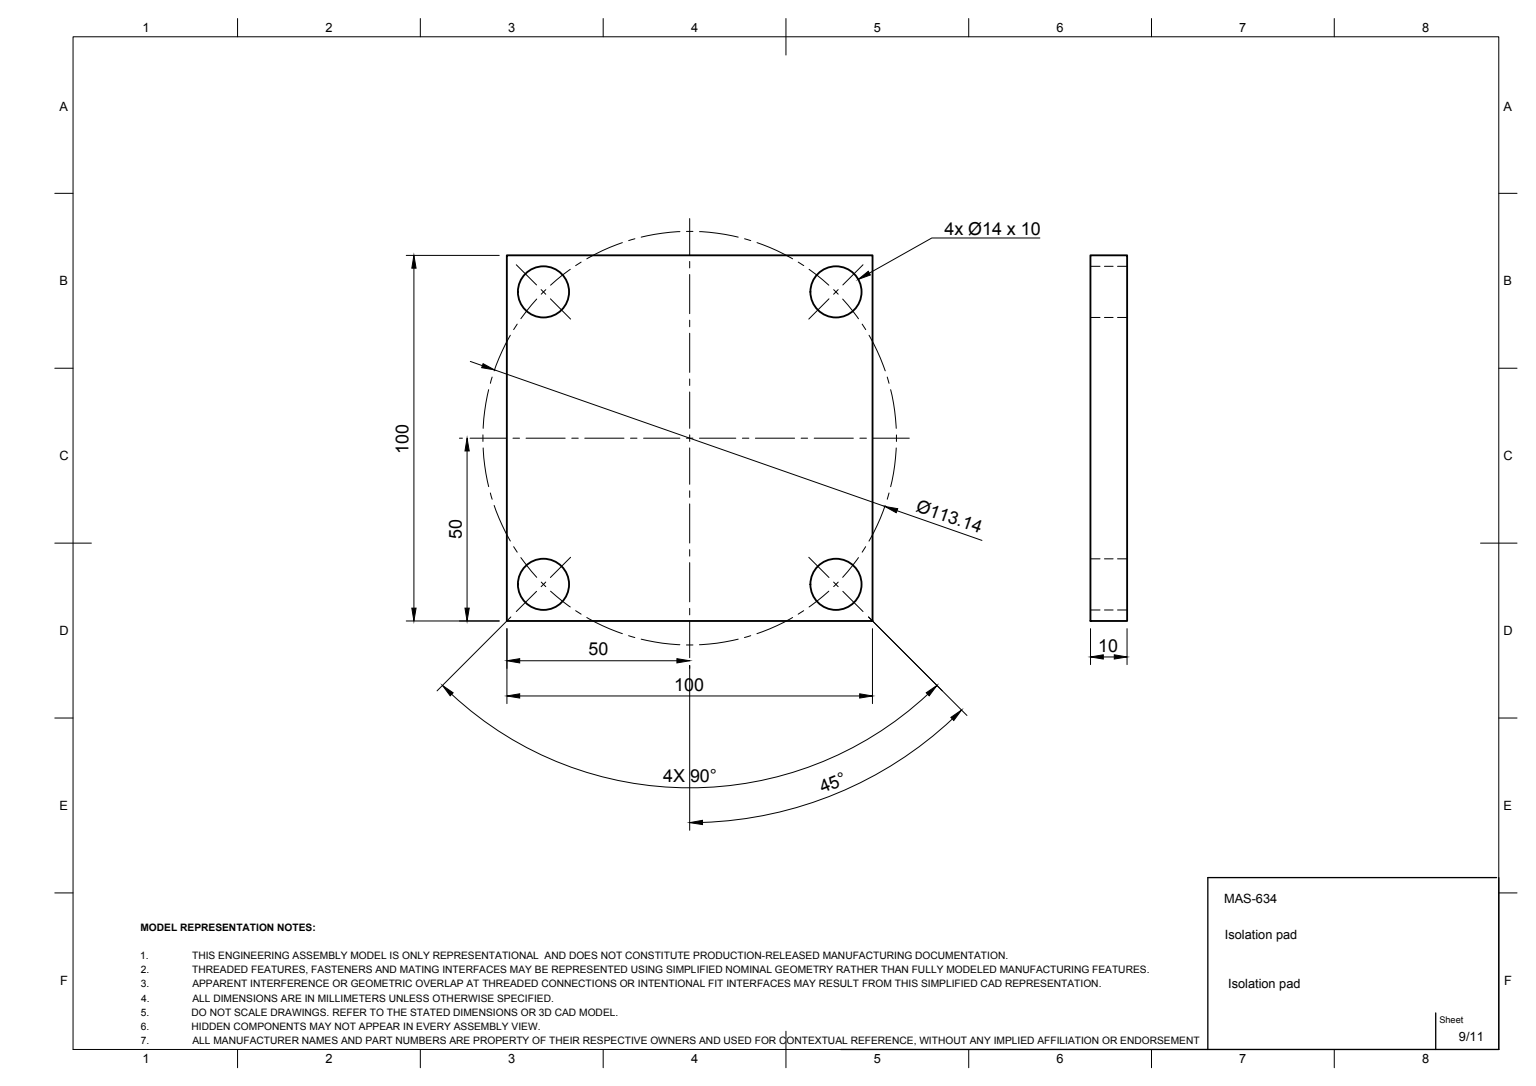
ISO-10303-21;
HEADER;
/* Generated by software containing ST-Developer
 * from STEP Tools, Inc. (www.steptools.com) 
 */

FILE_DESCRIPTION(
/* description */ ('Independent AHU equipment rack. Nominal800x600 frame on1000long40squa
re aluminum posts; two removable notched shelves; welded perimeter/cro
ss rails and rear gussets; two mounting channels; four isolation pads 
and anchor-ready feet. Imported native extrusion library retained and 
cut-length parameters customized per family. Shelf hardware uses model
ed M6 rivet nuts and screws. Weld design, floor anchors and load ratin
g require engineering selection.'),
/* implementation_level */ '2;1');

FILE_NAME(
/* name */ 'Isolation pad.step',
/* time_stamp */ '2026-11-07T19:04:45-08:00',
/* author */ (''),
/* organization */ (''),
/* preprocessor_version */ 'ST-DEVELOPER v20.2',
/* originating_system */ 'Autodesk Translation Framework v15.17.0.0',
/* authorisation */ '');

FILE_SCHEMA (('AUTOMOTIVE_DESIGN { 1 0 10303 214 3 1 1 }'));
ENDSEC;

DATA;
#10=MECHANICAL_DESIGN_GEOMETRIC_PRESENTATION_REPRESENTATION('',(#341),#9777);
#319=SHAPE_REPRESENTATION_RELATIONSHIP('SRR','None',#9863,#330);
#330=ADVANCED_BREP_SHAPE_REPRESENTATION('',(#352),#9772);
#341=STYLED_ITEM('',(#9926),#352);
#352=MANIFOLD_SOLID_BREP('Body1',#3846);
#395=FACE_BOUND('',#855,.T.);
#396=FACE_BOUND('',#856,.T.);
#397=FACE_BOUND('',#857,.T.);
#398=FACE_BOUND('',#858,.T.);
#399=FACE_BOUND('',#860,.T.);
#400=FACE_BOUND('',#861,.T.);
#401=FACE_BOUND('',#862,.T.);
#402=FACE_BOUND('',#863,.T.);
#470=PLANE('',#4197);
#471=PLANE('',#4198);
#472=PLANE('',#4199);
#473=PLANE('',#4200);
#474=PLANE('',#4201);
#475=PLANE('',#4202);
#610=FACE_OUTER_BOUND('',#846,.T.);
#611=FACE_OUTER_BOUND('',#847,.T.);
#612=FACE_OUTER_BOUND('',#848,.T.);
#613=FACE_OUTER_BOUND('',#849,.T.);
#614=FACE_OUTER_BOUND('',#850,.T.);
#615=FACE_OUTER_BOUND('',#851,.T.);
#616=FACE_OUTER_BOUND('',#852,.T.);
#617=FACE_OUTER_BOUND('',#853,.T.);
#618=FACE_OUTER_BOUND('',#854,.T.);
#619=FACE_OUTER_BOUND('',#859,.T.);
#846=EDGE_LOOP('',(#3091,#3092,#3093,#3094));
#847=EDGE_LOOP('',(#3095,#3096,#3097,#3098));
#848=EDGE_LOOP('',(#3099,#3100,#3101,#3102));
#849=EDGE_LOOP('',(#3103,#3104,#3105,#3106));
#850=EDGE_LOOP('',(#3107,#3108,#3109,#3110));
#851=EDGE_LOOP('',(#3111,#3112,#3113,#3114));
#852=EDGE_LOOP('',(#3115,#3116,#3117,#3118));
#853=EDGE_LOOP('',(#3119,#3120,#3121,#3122));
#854=EDGE_LOOP('',(#3123,#3124,#3125,#3126));
#855=EDGE_LOOP('',(#3127));
#856=EDGE_LOOP('',(#3128));
#857=EDGE_LOOP('',(#3129));
#858=EDGE_LOOP('',(#3130));
#859=EDGE_LOOP('',(#3131,#3132,#3133,#3134));
#860=EDGE_LOOP('',(#3135));
#861=EDGE_LOOP('',(#3136));
#862=EDGE_LOOP('',(#3137));
#863=EDGE_LOOP('',(#3138));
#1143=LINE('',#6003,#1436);
#1144=LINE('',#6009,#1437);
#1145=LINE('',#6015,#1438);
#1146=LINE('',#6021,#1439);
#1147=LINE('',#6026,#1440);
#1148=LINE('',#6028,#1441);
#1149=LINE('',#6030,#1442);
#1150=LINE('',#6031,#1443);
#1151=LINE('',#6034,#1444);
#1152=LINE('',#6036,#1445);
#1153=LINE('',#6037,#1446);
#1154=LINE('',#6040,#1447);
#1155=LINE('',#6042,#1448);
#1156=LINE('',#6043,#1449);
#1157=LINE('',#6045,#1450);
#1158=LINE('',#6046,#1451);
#1436=VECTOR('',#4972,7.);
#1437=VECTOR('',#4979,7.);
#1438=VECTOR('',#4986,7.);
#1439=VECTOR('',#4993,7.);
#1440=VECTOR('',#4998,10.);
#1441=VECTOR('',#4999,10.);
#1442=VECTOR('',#5000,10.);
#1443=VECTOR('',#5001,10.);
#1444=VECTOR('',#5004,10.);
#1445=VECTOR('',#5005,10.);
#1446=VECTOR('',#5006,10.);
#1447=VECTOR('',#5009,10.);
#1448=VECTOR('',#5010,10.);
#1449=VECTOR('',#5011,10.);
#1450=VECTOR('',#5014,10.);
#1451=VECTOR('',#5015,10.);
#1633=CIRCLE('',#4186,7.);
#1634=CIRCLE('',#4187,7.);
#1635=CIRCLE('',#4189,7.);
#1636=CIRCLE('',#4190,7.);
#1637=CIRCLE('',#4192,7.);
#1638=CIRCLE('',#4193,7.);
#1639=CIRCLE('',#4195,7.);
#1640=CIRCLE('',#4196,7.);
#1852=VERTEX_POINT('',#6000);
#1853=VERTEX_POINT('',#6002);
#1854=VERTEX_POINT('',#6006);
#1855=VERTEX_POINT('',#6008);
#1856=VERTEX_POINT('',#6012);
#1857=VERTEX_POINT('',#6014);
#1858=VERTEX_POINT('',#6018);
#1859=VERTEX_POINT('',#6020);
#1860=VERTEX_POINT('',#6024);
#1861=VERTEX_POINT('',#6025);
#1862=VERTEX_POINT('',#6027);
#1863=VERTEX_POINT('',#6029);
#1864=VERTEX_POINT('',#6033);
#1865=VERTEX_POINT('',#6035);
#1866=VERTEX_POINT('',#6039);
#1867=VERTEX_POINT('',#6041);
#2290=EDGE_CURVE('',#1852,#1852,#1633,.T.);
#2291=EDGE_CURVE('',#1852,#1853,#1143,.T.);
#2292=EDGE_CURVE('',#1853,#1853,#1634,.T.);
#2293=EDGE_CURVE('',#1854,#1854,#1635,.T.);
#2294=EDGE_CURVE('',#1854,#1855,#1144,.T.);
#2295=EDGE_CURVE('',#1855,#1855,#1636,.T.);
#2296=EDGE_CURVE('',#1856,#1856,#1637,.T.);
#2297=EDGE_CURVE('',#1856,#1857,#1145,.T.);
#2298=EDGE_CURVE('',#1857,#1857,#1638,.T.);
#2299=EDGE_CURVE('',#1858,#1858,#1639,.T.);
#2300=EDGE_CURVE('',#1858,#1859,#1146,.T.);
#2301=EDGE_CURVE('',#1859,#1859,#1640,.T.);
#2302=EDGE_CURVE('',#1860,#1861,#1147,.T.);
#2303=EDGE_CURVE('',#1861,#1862,#1148,.T.);
#2304=EDGE_CURVE('',#1863,#1862,#1149,.T.);
#2305=EDGE_CURVE('',#1860,#1863,#1150,.T.);
#2306=EDGE_CURVE('',#1864,#1860,#1151,.T.);
#2307=EDGE_CURVE('',#1865,#1863,#1152,.T.);
#2308=EDGE_CURVE('',#1864,#1865,#1153,.T.);
#2309=EDGE_CURVE('',#1866,#1864,#1154,.T.);
#2310=EDGE_CURVE('',#1867,#1865,#1155,.T.);
#2311=EDGE_CURVE('',#1866,#1867,#1156,.T.);
#2312=EDGE_CURVE('',#1861,#1866,#1157,.T.);
#2313=EDGE_CURVE('',#1862,#1867,#1158,.T.);
#3091=ORIENTED_EDGE('',*,*,#2290,.F.);
#3092=ORIENTED_EDGE('',*,*,#2291,.T.);
#3093=ORIENTED_EDGE('',*,*,#2292,.F.);
#3094=ORIENTED_EDGE('',*,*,#2291,.F.);
#3095=ORIENTED_EDGE('',*,*,#2293,.F.);
#3096=ORIENTED_EDGE('',*,*,#2294,.T.);
#3097=ORIENTED_EDGE('',*,*,#2295,.F.);
#3098=ORIENTED_EDGE('',*,*,#2294,.F.);
#3099=ORIENTED_EDGE('',*,*,#2296,.F.);
#3100=ORIENTED_EDGE('',*,*,#2297,.T.);
#3101=ORIENTED_EDGE('',*,*,#2298,.F.);
#3102=ORIENTED_EDGE('',*,*,#2297,.F.);
#3103=ORIENTED_EDGE('',*,*,#2299,.F.);
#3104=ORIENTED_EDGE('',*,*,#2300,.T.);
#3105=ORIENTED_EDGE('',*,*,#2301,.F.);
#3106=ORIENTED_EDGE('',*,*,#2300,.F.);
#3107=ORIENTED_EDGE('',*,*,#2302,.T.);
#3108=ORIENTED_EDGE('',*,*,#2303,.T.);
#3109=ORIENTED_EDGE('',*,*,#2304,.F.);
#3110=ORIENTED_EDGE('',*,*,#2305,.F.);
#3111=ORIENTED_EDGE('',*,*,#2306,.T.);
#3112=ORIENTED_EDGE('',*,*,#2305,.T.);
#3113=ORIENTED_EDGE('',*,*,#2307,.F.);
#3114=ORIENTED_EDGE('',*,*,#2308,.F.);
#3115=ORIENTED_EDGE('',*,*,#2309,.T.);
#3116=ORIENTED_EDGE('',*,*,#2308,.T.);
#3117=ORIENTED_EDGE('',*,*,#2310,.F.);
#3118=ORIENTED_EDGE('',*,*,#2311,.F.);
#3119=ORIENTED_EDGE('',*,*,#2312,.T.);
#3120=ORIENTED_EDGE('',*,*,#2311,.T.);
#3121=ORIENTED_EDGE('',*,*,#2313,.F.);
#3122=ORIENTED_EDGE('',*,*,#2303,.F.);
#3123=ORIENTED_EDGE('',*,*,#2313,.T.);
#3124=ORIENTED_EDGE('',*,*,#2310,.T.);
#3125=ORIENTED_EDGE('',*,*,#2307,.T.);
#3126=ORIENTED_EDGE('',*,*,#2304,.T.);
#3127=ORIENTED_EDGE('',*,*,#2290,.T.);
#3128=ORIENTED_EDGE('',*,*,#2293,.T.);
#3129=ORIENTED_EDGE('',*,*,#2296,.T.);
#3130=ORIENTED_EDGE('',*,*,#2299,.T.);
#3131=ORIENTED_EDGE('',*,*,#2312,.F.);
#3132=ORIENTED_EDGE('',*,*,#2302,.F.);
#3133=ORIENTED_EDGE('',*,*,#2306,.F.);
#3134=ORIENTED_EDGE('',*,*,#2309,.F.);
#3135=ORIENTED_EDGE('',*,*,#2292,.T.);
#3136=ORIENTED_EDGE('',*,*,#2295,.T.);
#3137=ORIENTED_EDGE('',*,*,#2298,.T.);
#3138=ORIENTED_EDGE('',*,*,#2301,.T.);
#3589=CYLINDRICAL_SURFACE('',#4185,7.);
#3590=CYLINDRICAL_SURFACE('',#4188,7.);
#3591=CYLINDRICAL_SURFACE('',#4191,7.);
#3592=CYLINDRICAL_SURFACE('',#4194,7.);
#3750=ADVANCED_FACE('',(#610),#3589,.F.);
#3751=ADVANCED_FACE('',(#611),#3590,.F.);
#3752=ADVANCED_FACE('',(#612),#3591,.F.);
#3753=ADVANCED_FACE('',(#613),#3592,.F.);
#3754=ADVANCED_FACE('',(#614),#470,.T.);
#3755=ADVANCED_FACE('',(#615),#471,.T.);
#3756=ADVANCED_FACE('',(#616),#472,.T.);
#3757=ADVANCED_FACE('',(#617),#473,.T.);
#3758=ADVANCED_FACE('',(#618,#395,#396,#397,#398),#474,.T.);
#3759=ADVANCED_FACE('',(#619,#399,#400,#401,#402),#475,.F.);
#3846=CLOSED_SHELL('',(#3750,#3751,#3752,#3753,#3754,#3755,#3756,#3757,
#3758,#3759));
#4184=AXIS2_PLACEMENT_3D('',#5998,#4966,#4967);
#4185=AXIS2_PLACEMENT_3D('',#5999,#4968,#4969);
#4186=AXIS2_PLACEMENT_3D('',#6001,#4970,#4971);
#4187=AXIS2_PLACEMENT_3D('',#6004,#4973,#4974);
#4188=AXIS2_PLACEMENT_3D('',#6005,#4975,#4976);
#4189=AXIS2_PLACEMENT_3D('',#6007,#4977,#4978);
#4190=AXIS2_PLACEMENT_3D('',#6010,#4980,#4981);
#4191=AXIS2_PLACEMENT_3D('',#6011,#4982,#4983);
#4192=AXIS2_PLACEMENT_3D('',#6013,#4984,#4985);
#4193=AXIS2_PLACEMENT_3D('',#6016,#4987,#4988);
#4194=AXIS2_PLACEMENT_3D('',#6017,#4989,#4990);
#4195=AXIS2_PLACEMENT_3D('',#6019,#4991,#4992);
#4196=AXIS2_PLACEMENT_3D('',#6022,#4994,#4995);
#4197=AXIS2_PLACEMENT_3D('',#6023,#4996,#4997);
#4198=AXIS2_PLACEMENT_3D('',#6032,#5002,#5003);
#4199=AXIS2_PLACEMENT_3D('',#6038,#5007,#5008);
#4200=AXIS2_PLACEMENT_3D('',#6044,#5012,#5013);
#4201=AXIS2_PLACEMENT_3D('',#6047,#5016,#5017);
#4202=AXIS2_PLACEMENT_3D('',#6048,#5018,#5019);
#4966=DIRECTION('axis',(0.,0.,1.));
#4967=DIRECTION('refdir',(1.,0.,0.));
#4968=DIRECTION('center_axis',(0.,0.,-1.));
#4969=DIRECTION('ref_axis',(1.,0.,0.));
#4970=DIRECTION('center_axis',(0.,0.,-1.));
#4971=DIRECTION('ref_axis',(1.,0.,0.));
#4972=DIRECTION('',(0.,0.,-1.));
#4973=DIRECTION('center_axis',(0.,0.,1.));
#4974=DIRECTION('ref_axis',(1.,0.,0.));
#4975=DIRECTION('center_axis',(0.,0.,-1.));
#4976=DIRECTION('ref_axis',(1.,0.,0.));
#4977=DIRECTION('center_axis',(0.,0.,-1.));
#4978=DIRECTION('ref_axis',(1.,0.,0.));
#4979=DIRECTION('',(0.,0.,-1.));
#4980=DIRECTION('center_axis',(0.,0.,1.));
#4981=DIRECTION('ref_axis',(1.,0.,0.));
#4982=DIRECTION('center_axis',(0.,0.,-1.));
#4983=DIRECTION('ref_axis',(1.,0.,0.));
#4984=DIRECTION('center_axis',(0.,0.,-1.));
#4985=DIRECTION('ref_axis',(1.,0.,0.));
#4986=DIRECTION('',(0.,0.,-1.));
#4987=DIRECTION('center_axis',(0.,0.,1.));
#4988=DIRECTION('ref_axis',(1.,0.,0.));
#4989=DIRECTION('center_axis',(0.,0.,-1.));
#4990=DIRECTION('ref_axis',(1.,0.,0.));
#4991=DIRECTION('center_axis',(0.,0.,-1.));
#4992=DIRECTION('ref_axis',(1.,0.,0.));
#4993=DIRECTION('',(0.,0.,-1.));
#4994=DIRECTION('center_axis',(0.,0.,1.));
#4995=DIRECTION('ref_axis',(1.,0.,0.));
#4996=DIRECTION('center_axis',(0.,1.,0.));
#4997=DIRECTION('ref_axis',(-1.,0.,0.));
#4998=DIRECTION('',(-1.,0.,0.));
#4999=DIRECTION('',(0.,0.,1.));
#5000=DIRECTION('',(-1.,0.,0.));
#5001=DIRECTION('',(0.,0.,1.));
#5002=DIRECTION('center_axis',(1.,0.,0.));
#5003=DIRECTION('ref_axis',(0.,1.,0.));
#5004=DIRECTION('',(0.,1.,0.));
#5005=DIRECTION('',(0.,1.,0.));
#5006=DIRECTION('',(0.,0.,1.));
#5007=DIRECTION('center_axis',(0.,-1.,0.));
#5008=DIRECTION('ref_axis',(1.,0.,0.));
#5009=DIRECTION('',(1.,0.,0.));
#5010=DIRECTION('',(1.,0.,0.));
#5011=DIRECTION('',(0.,0.,1.));
#5012=DIRECTION('center_axis',(-1.,0.,0.));
#5013=DIRECTION('ref_axis',(0.,-1.,0.));
#5014=DIRECTION('',(0.,-1.,0.));
#5015=DIRECTION('',(0.,-1.,0.));
#5016=DIRECTION('center_axis',(0.,0.,1.));
#5017=DIRECTION('ref_axis',(1.,0.,0.));
#5018=DIRECTION('center_axis',(0.,0.,1.));
#5019=DIRECTION('ref_axis',(1.,0.,0.));
#5998=CARTESIAN_POINT('',(0.,0.,0.));
#5999=CARTESIAN_POINT('Origin',(40.,-40.,5.));
#6000=CARTESIAN_POINT('',(33.,-40.,10.));
#6001=CARTESIAN_POINT('Origin',(40.,-40.,10.));
#6002=CARTESIAN_POINT('',(33.,-40.,0.));
#6003=CARTESIAN_POINT('',(33.,-40.,5.));
#6004=CARTESIAN_POINT('Origin',(40.,-40.,0.));
#6005=CARTESIAN_POINT('Origin',(-40.,-40.,5.));
#6006=CARTESIAN_POINT('',(-47.,-40.,10.));
#6007=CARTESIAN_POINT('Origin',(-40.,-40.,10.));
#6008=CARTESIAN_POINT('',(-47.,-40.,0.));
#6009=CARTESIAN_POINT('',(-47.,-40.,5.));
#6010=CARTESIAN_POINT('Origin',(-40.,-40.,0.));
#6011=CARTESIAN_POINT('Origin',(-40.,40.,5.));
#6012=CARTESIAN_POINT('',(-47.,40.,10.));
#6013=CARTESIAN_POINT('Origin',(-40.,40.,10.));
#6014=CARTESIAN_POINT('',(-47.,40.,0.));
#6015=CARTESIAN_POINT('',(-47.,40.,5.));
#6016=CARTESIAN_POINT('Origin',(-40.,40.,0.));
#6017=CARTESIAN_POINT('Origin',(40.,40.,5.));
#6018=CARTESIAN_POINT('',(33.,40.,10.));
#6019=CARTESIAN_POINT('Origin',(40.,40.,10.));
#6020=CARTESIAN_POINT('',(33.,40.,0.));
#6021=CARTESIAN_POINT('',(33.,40.,5.));
#6022=CARTESIAN_POINT('Origin',(40.,40.,0.));
#6023=CARTESIAN_POINT('Origin',(50.,50.,0.));
#6024=CARTESIAN_POINT('',(50.,50.,0.));
#6025=CARTESIAN_POINT('',(-50.,50.,0.));
#6026=CARTESIAN_POINT('',(50.,50.,0.));
#6027=CARTESIAN_POINT('',(-50.,50.,10.));
#6028=CARTESIAN_POINT('',(-50.,50.,0.));
#6029=CARTESIAN_POINT('',(50.,50.,10.));
#6030=CARTESIAN_POINT('',(50.,50.,10.));
#6031=CARTESIAN_POINT('',(50.,50.,0.));
#6032=CARTESIAN_POINT('Origin',(50.,-50.,0.));
#6033=CARTESIAN_POINT('',(50.,-50.,0.));
#6034=CARTESIAN_POINT('',(50.,-50.,0.));
#6035=CARTESIAN_POINT('',(50.,-50.,10.));
#6036=CARTESIAN_POINT('',(50.,-50.,10.));
#6037=CARTESIAN_POINT('',(50.,-50.,0.));
#6038=CARTESIAN_POINT('Origin',(-50.,-50.,0.));
#6039=CARTESIAN_POINT('',(-50.,-50.,0.));
#6040=CARTESIAN_POINT('',(-50.,-50.,0.));
#6041=CARTESIAN_POINT('',(-50.,-50.,10.));
#6042=CARTESIAN_POINT('',(-50.,-50.,10.));
#6043=CARTESIAN_POINT('',(-50.,-50.,0.));
#6044=CARTESIAN_POINT('Origin',(-50.,50.,0.));
#6045=CARTESIAN_POINT('',(-50.,50.,0.));
#6046=CARTESIAN_POINT('',(-50.,50.,10.));
#6047=CARTESIAN_POINT('Origin',(0.,0.,10.));
#6048=CARTESIAN_POINT('Origin',(0.,0.,0.));
#9759=UNCERTAINTY_MEASURE_WITH_UNIT(LENGTH_MEASURE(0.01),#9778,
'DISTANCE_ACCURACY_VALUE',
'Maximum model space distance between geometric entities at asserted c
onnectivities');
#9764=UNCERTAINTY_MEASURE_WITH_UNIT(LENGTH_MEASURE(0.01),#9778,
'DISTANCE_ACCURACY_VALUE',
'Maximum model space distance between geometric entities at asserted c
onnectivities');
#9772=(
GEOMETRIC_REPRESENTATION_CONTEXT(3)
GLOBAL_UNCERTAINTY_ASSIGNED_CONTEXT((#9759))
GLOBAL_UNIT_ASSIGNED_CONTEXT((#9778,#9780,#9781))
REPRESENTATION_CONTEXT('','3D')
);
#9777=(
GEOMETRIC_REPRESENTATION_CONTEXT(3)
GLOBAL_UNCERTAINTY_ASSIGNED_CONTEXT((#9764))
GLOBAL_UNIT_ASSIGNED_CONTEXT((#9778,#9780,#9781))
REPRESENTATION_CONTEXT('','3D')
);
#9778=(
LENGTH_UNIT()
NAMED_UNIT(*)
SI_UNIT(.MILLI.,.METRE.)
);
#9780=(
NAMED_UNIT(*)
PLANE_ANGLE_UNIT()
SI_UNIT($,.RADIAN.)
);
#9781=(
NAMED_UNIT(*)
SI_UNIT($,.STERADIAN.)
SOLID_ANGLE_UNIT()
);
#9789=SHAPE_DEFINITION_REPRESENTATION(#9801,#9863);
#9801=PRODUCT_DEFINITION_SHAPE('',$,#9876);
#9863=SHAPE_REPRESENTATION('',(#4184),#9772);
#9868=PRODUCT_DEFINITION_CONTEXT('part definition',#9906,'design');
#9876=PRODUCT_DEFINITION('Isolation pad','Isolation pad',#9888,#9868);
#9888=PRODUCT_DEFINITION_FORMATION('',$,#9915);
#9906=APPLICATION_CONTEXT(
'Core Data for Automotive Mechanical Design Process');
#9907=PRODUCT_CONTEXT('part definition',#9906,'mechanical');
#9915=PRODUCT('Isolation pad','Isolation pad',$,(#9907));
#9926=PRESENTATION_STYLE_ASSIGNMENT((#9937));
#9937=SURFACE_STYLE_USAGE(.BOTH.,#9948);
#9948=SURFACE_SIDE_STYLE('',(#9959));
#9959=SURFACE_STYLE_FILL_AREA(#9970);
#9970=FILL_AREA_STYLE('Pad charcoal',(#9981));
#9981=FILL_AREA_STYLE_COLOUR('Pad charcoal',#9992);
#9992=COLOUR_RGB('Pad charcoal',0.164705882352941,0.184313725490196,0.211764705882353);
ENDSEC;
END-ISO-10303-21;
